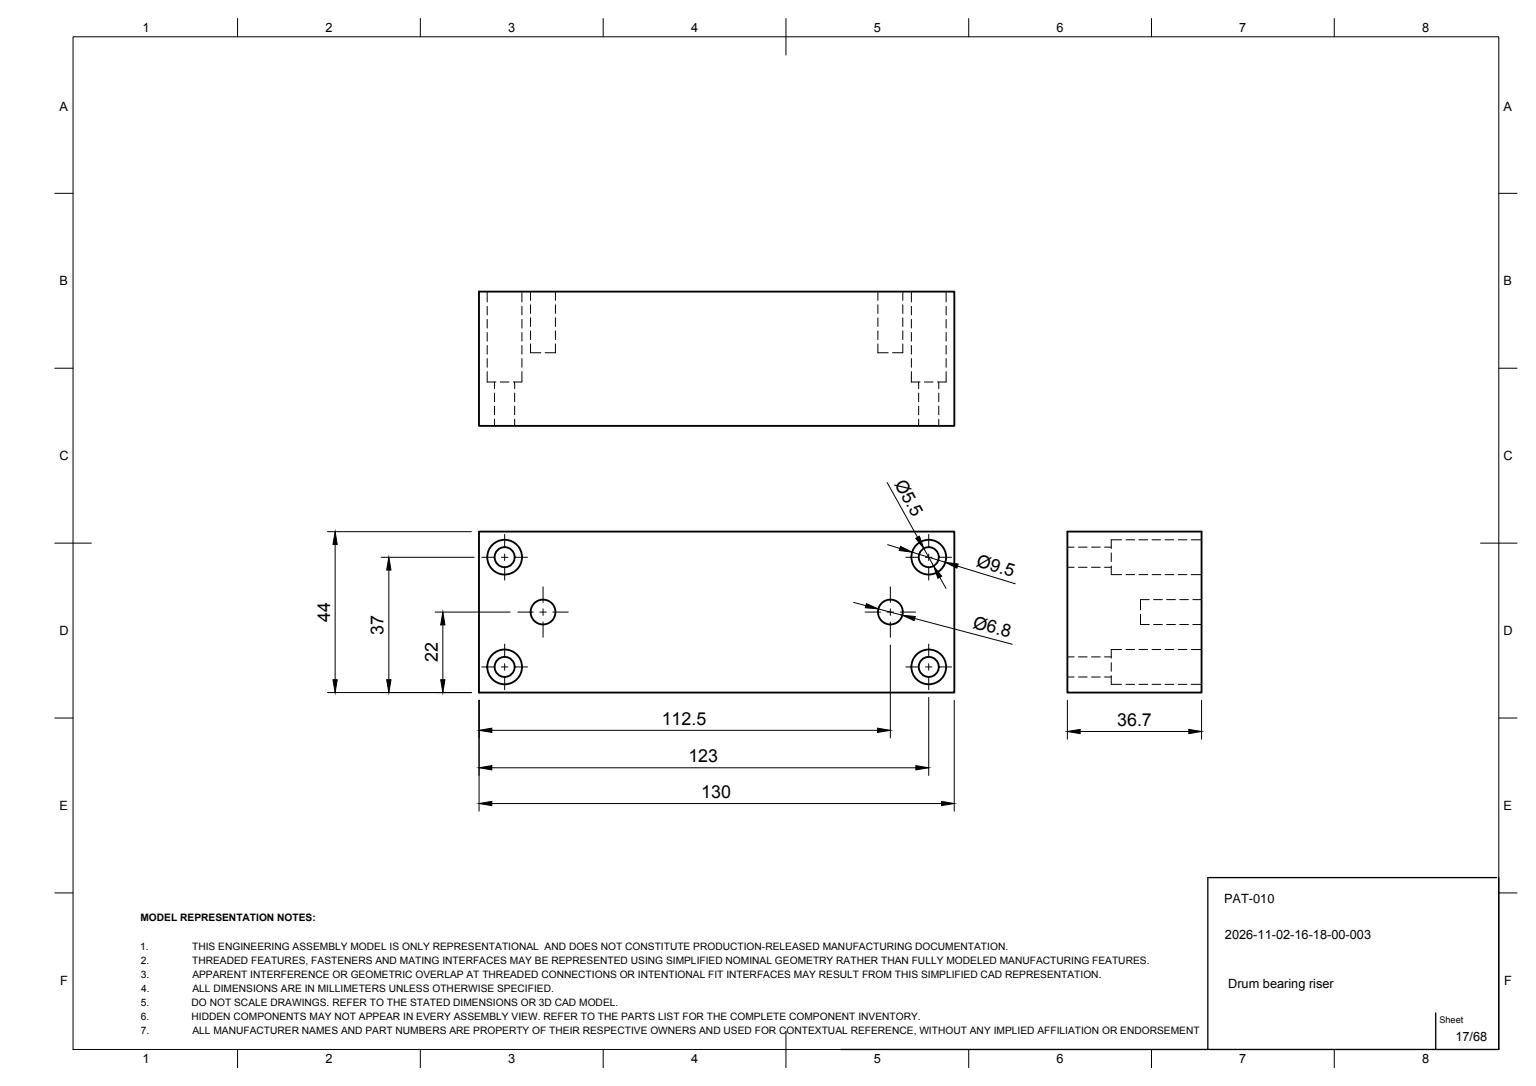
ISO-10303-21;
HEADER;
/* Generated by software containing ST-Developer
 * from STEP Tools, Inc. (www.steptools.com) 
 */

FILE_DESCRIPTION(
/* description */ ('Belt conveyor head drive unit'),
/* implementation_level */ '2;1');

FILE_NAME(
/* name */ 'Drum bearing riser.step',
/* time_stamp */ '2026-10-28T03:26:19-07:00',
/* author */ (''),
/* organization */ (''),
/* preprocessor_version */ 'ST-DEVELOPER v20.2',
/* originating_system */ 'Autodesk Translation Framework v15.17.0.0',
/* authorisation */ '');

FILE_SCHEMA (('AUTOMOTIVE_DESIGN { 1 0 10303 214 3 1 1 }'));
ENDSEC;

DATA;
#10=MECHANICAL_DESIGN_GEOMETRIC_PRESENTATION_REPRESENTATION('',(#863),#27069);
#725=SHAPE_REPRESENTATION_RELATIONSHIP('SRR','None',#27369,#794);
#794=ADVANCED_BREP_SHAPE_REPRESENTATION('',(#948),#27011);
#863=STYLED_ITEM('',(#27797),#948);
#948=MANIFOLD_SOLID_BREP('Body1',#13728);
#1093=FACE_BOUND('',#2714,.T.);
#1094=FACE_BOUND('',#2718,.T.);
#1095=FACE_BOUND('',#2722,.T.);
#1096=FACE_BOUND('',#2726,.T.);
#1097=FACE_BOUND('',#2737,.T.);
#1098=FACE_BOUND('',#2738,.T.);
#1099=FACE_BOUND('',#2739,.T.);
#1100=FACE_BOUND('',#2740,.T.);
#1101=FACE_BOUND('',#2741,.T.);
#1102=FACE_BOUND('',#2742,.T.);
#1103=FACE_BOUND('',#2744,.T.);
#1104=FACE_BOUND('',#2745,.T.);
#1105=FACE_BOUND('',#2746,.T.);
#1106=FACE_BOUND('',#2747,.T.);
#1373=PLANE('',#14998);
#1374=PLANE('',#15005);
#1375=PLANE('',#15012);
#1376=PLANE('',#15019);
#1377=PLANE('',#15026);
#1378=PLANE('',#15030);
#1379=PLANE('',#15031);
#1380=PLANE('',#15032);
#1381=PLANE('',#15033);
#1382=PLANE('',#15034);
#1383=PLANE('',#15035);
#1384=PLANE('',#15036);
#1831=FACE_OUTER_BOUND('',#2712,.T.);
#1832=FACE_OUTER_BOUND('',#2713,.T.);
#1833=FACE_OUTER_BOUND('',#2715,.T.);
#1834=FACE_OUTER_BOUND('',#2716,.T.);
#1835=FACE_OUTER_BOUND('',#2717,.T.);
#1836=FACE_OUTER_BOUND('',#2719,.T.);
#1837=FACE_OUTER_BOUND('',#2720,.T.);
#1838=FACE_OUTER_BOUND('',#2721,.T.);
#1839=FACE_OUTER_BOUND('',#2723,.T.);
#1840=FACE_OUTER_BOUND('',#2724,.T.);
#1841=FACE_OUTER_BOUND('',#2725,.T.);
#1842=FACE_OUTER_BOUND('',#2727,.T.);
#1843=FACE_OUTER_BOUND('',#2728,.T.);
#1844=FACE_OUTER_BOUND('',#2729,.T.);
#1845=FACE_OUTER_BOUND('',#2730,.T.);
#1846=FACE_OUTER_BOUND('',#2731,.T.);
#1847=FACE_OUTER_BOUND('',#2732,.T.);
#1848=FACE_OUTER_BOUND('',#2733,.T.);
#1849=FACE_OUTER_BOUND('',#2734,.T.);
#1850=FACE_OUTER_BOUND('',#2735,.T.);
#1851=FACE_OUTER_BOUND('',#2736,.T.);
#1852=FACE_OUTER_BOUND('',#2743,.T.);
#2712=EDGE_LOOP('',(#9864,#9865,#9866,#9867));
#2713=EDGE_LOOP('',(#9868));
#2714=EDGE_LOOP('',(#9869));
#2715=EDGE_LOOP('',(#9870,#9871,#9872,#9873));
#2716=EDGE_LOOP('',(#9874,#9875,#9876,#9877));
#2717=EDGE_LOOP('',(#9878));
#2718=EDGE_LOOP('',(#9879));
#2719=EDGE_LOOP('',(#9880,#9881,#9882,#9883));
#2720=EDGE_LOOP('',(#9884,#9885,#9886,#9887));
#2721=EDGE_LOOP('',(#9888));
#2722=EDGE_LOOP('',(#9889));
#2723=EDGE_LOOP('',(#9890,#9891,#9892,#9893));
#2724=EDGE_LOOP('',(#9894,#9895,#9896,#9897));
#2725=EDGE_LOOP('',(#9898));
#2726=EDGE_LOOP('',(#9899));
#2727=EDGE_LOOP('',(#9900,#9901,#9902,#9903));
#2728=EDGE_LOOP('',(#9904,#9905,#9906,#9907));
#2729=EDGE_LOOP('',(#9908));
#2730=EDGE_LOOP('',(#9909,#9910,#9911,#9912));
#2731=EDGE_LOOP('',(#9913));
#2732=EDGE_LOOP('',(#9914,#9915,#9916,#9917));
#2733=EDGE_LOOP('',(#9918,#9919,#9920,#9921));
#2734=EDGE_LOOP('',(#9922,#9923,#9924,#9925));
#2735=EDGE_LOOP('',(#9926,#9927,#9928,#9929));
#2736=EDGE_LOOP('',(#9930,#9931,#9932,#9933));
#2737=EDGE_LOOP('',(#9934));
#2738=EDGE_LOOP('',(#9935));
#2739=EDGE_LOOP('',(#9936));
#2740=EDGE_LOOP('',(#9937));
#2741=EDGE_LOOP('',(#9938));
#2742=EDGE_LOOP('',(#9939));
#2743=EDGE_LOOP('',(#9940,#9941,#9942,#9943));
#2744=EDGE_LOOP('',(#9944));
#2745=EDGE_LOOP('',(#9945));
#2746=EDGE_LOOP('',(#9946));
#2747=EDGE_LOOP('',(#9947));
#3735=LINE('',#21946,#4527);
#3736=LINE('',#21954,#4528);
#3737=LINE('',#21959,#4529);
#3738=LINE('',#21967,#4530);
#3739=LINE('',#21972,#4531);
#3740=LINE('',#21980,#4532);
#3741=LINE('',#21985,#4533);
#3742=LINE('',#21993,#4534);
#3743=LINE('',#21998,#4535);
#3744=LINE('',#22005,#4536);
#3745=LINE('',#22011,#4537);
#3746=LINE('',#22013,#4538);
#3747=LINE('',#22015,#4539);
#3748=LINE('',#22016,#4540);
#3749=LINE('',#22019,#4541);
#3750=LINE('',#22021,#4542);
#3751=LINE('',#22022,#4543);
#3752=LINE('',#22025,#4544);
#3753=LINE('',#22027,#4545);
#3754=LINE('',#22028,#4546);
#3755=LINE('',#22030,#4547);
#3756=LINE('',#22031,#4548);
#4527=VECTOR('',#17541,0.475);
#4528=VECTOR('',#17552,0.275);
#4529=VECTOR('',#17557,0.475);
#4530=VECTOR('',#17568,0.275);
#4531=VECTOR('',#17573,0.475);
#4532=VECTOR('',#17584,0.275);
#4533=VECTOR('',#17589,0.475);
#4534=VECTOR('',#17600,0.275);
#4535=VECTOR('',#17605,0.34);
#4536=VECTOR('',#17614,0.34);
#4537=VECTOR('',#17621,1.);
#4538=VECTOR('',#17622,1.);
#4539=VECTOR('',#17623,1.);
#4540=VECTOR('',#17624,1.);
#4541=VECTOR('',#17627,1.);
#4542=VECTOR('',#17628,1.);
#4543=VECTOR('',#17629,1.);
#4544=VECTOR('',#17632,1.);
#4545=VECTOR('',#17633,1.);
#4546=VECTOR('',#17634,1.);
#4547=VECTOR('',#17637,1.);
#4548=VECTOR('',#17638,1.);
#5298=CIRCLE('',#14996,0.475);
#5299=CIRCLE('',#14997,0.475);
#5300=CIRCLE('',#14999,0.275);
#5301=CIRCLE('',#15001,0.275);
#5302=CIRCLE('',#15003,0.475);
#5303=CIRCLE('',#15004,0.475);
#5304=CIRCLE('',#15006,0.275);
#5305=CIRCLE('',#15008,0.275);
#5306=CIRCLE('',#15010,0.475);
#5307=CIRCLE('',#15011,0.475);
#5308=CIRCLE('',#15013,0.275);
#5309=CIRCLE('',#15015,0.275);
#5310=CIRCLE('',#15017,0.475);
#5311=CIRCLE('',#15018,0.475);
#5312=CIRCLE('',#15020,0.275);
#5313=CIRCLE('',#15022,0.275);
#5314=CIRCLE('',#15024,0.34);
#5315=CIRCLE('',#15025,0.34);
#5316=CIRCLE('',#15028,0.34);
#5317=CIRCLE('',#15029,0.34);
#6255=VERTEX_POINT('',#21943);
#6256=VERTEX_POINT('',#21945);
#6257=VERTEX_POINT('',#21949);
#6258=VERTEX_POINT('',#21952);
#6259=VERTEX_POINT('',#21956);
#6260=VERTEX_POINT('',#21958);
#6261=VERTEX_POINT('',#21962);
#6262=VERTEX_POINT('',#21965);
#6263=VERTEX_POINT('',#21969);
#6264=VERTEX_POINT('',#21971);
#6265=VERTEX_POINT('',#21975);
#6266=VERTEX_POINT('',#21978);
#6267=VERTEX_POINT('',#21982);
#6268=VERTEX_POINT('',#21984);
#6269=VERTEX_POINT('',#21988);
#6270=VERTEX_POINT('',#21991);
#6271=VERTEX_POINT('',#21995);
#6272=VERTEX_POINT('',#21997);
#6273=VERTEX_POINT('',#22002);
#6274=VERTEX_POINT('',#22004);
#6275=VERTEX_POINT('',#22009);
#6276=VERTEX_POINT('',#22010);
#6277=VERTEX_POINT('',#22012);
#6278=VERTEX_POINT('',#22014);
#6279=VERTEX_POINT('',#22018);
#6280=VERTEX_POINT('',#22020);
#6281=VERTEX_POINT('',#22024);
#6282=VERTEX_POINT('',#22026);
#7624=EDGE_CURVE('',#6255,#6255,#5298,.T.);
#7625=EDGE_CURVE('',#6255,#6256,#3735,.T.);
#7626=EDGE_CURVE('',#6256,#6256,#5299,.T.);
#7627=EDGE_CURVE('',#6257,#6257,#5300,.T.);
#7628=EDGE_CURVE('',#6258,#6258,#5301,.T.);
#7629=EDGE_CURVE('',#6258,#6257,#3736,.T.);
#7630=EDGE_CURVE('',#6259,#6259,#5302,.T.);
#7631=EDGE_CURVE('',#6259,#6260,#3737,.T.);
#7632=EDGE_CURVE('',#6260,#6260,#5303,.T.);
#7633=EDGE_CURVE('',#6261,#6261,#5304,.T.);
#7634=EDGE_CURVE('',#6262,#6262,#5305,.T.);
#7635=EDGE_CURVE('',#6262,#6261,#3738,.T.);
#7636=EDGE_CURVE('',#6263,#6263,#5306,.T.);
#7637=EDGE_CURVE('',#6263,#6264,#3739,.T.);
#7638=EDGE_CURVE('',#6264,#6264,#5307,.T.);
#7639=EDGE_CURVE('',#6265,#6265,#5308,.T.);
#7640=EDGE_CURVE('',#6266,#6266,#5309,.T.);
#7641=EDGE_CURVE('',#6266,#6265,#3740,.T.);
#7642=EDGE_CURVE('',#6267,#6267,#5310,.T.);
#7643=EDGE_CURVE('',#6267,#6268,#3741,.T.);
#7644=EDGE_CURVE('',#6268,#6268,#5311,.T.);
#7645=EDGE_CURVE('',#6269,#6269,#5312,.T.);
#7646=EDGE_CURVE('',#6270,#6270,#5313,.T.);
#7647=EDGE_CURVE('',#6270,#6269,#3742,.T.);
#7648=EDGE_CURVE('',#6271,#6271,#5314,.T.);
#7649=EDGE_CURVE('',#6271,#6272,#3743,.T.);
#7650=EDGE_CURVE('',#6272,#6272,#5315,.T.);
#7651=EDGE_CURVE('',#6273,#6273,#5316,.T.);
#7652=EDGE_CURVE('',#6273,#6274,#3744,.T.);
#7653=EDGE_CURVE('',#6274,#6274,#5317,.T.);
#7654=EDGE_CURVE('',#6275,#6276,#3745,.T.);
#7655=EDGE_CURVE('',#6276,#6277,#3746,.T.);
#7656=EDGE_CURVE('',#6278,#6277,#3747,.T.);
#7657=EDGE_CURVE('',#6275,#6278,#3748,.T.);
#7658=EDGE_CURVE('',#6279,#6275,#3749,.T.);
#7659=EDGE_CURVE('',#6280,#6278,#3750,.T.);
#7660=EDGE_CURVE('',#6279,#6280,#3751,.T.);
#7661=EDGE_CURVE('',#6281,#6279,#3752,.T.);
#7662=EDGE_CURVE('',#6282,#6280,#3753,.T.);
#7663=EDGE_CURVE('',#6281,#6282,#3754,.T.);
#7664=EDGE_CURVE('',#6276,#6281,#3755,.T.);
#7665=EDGE_CURVE('',#6277,#6282,#3756,.T.);
#9864=ORIENTED_EDGE('',*,*,#7624,.F.);
#9865=ORIENTED_EDGE('',*,*,#7625,.T.);
#9866=ORIENTED_EDGE('',*,*,#7626,.F.);
#9867=ORIENTED_EDGE('',*,*,#7625,.F.);
#9868=ORIENTED_EDGE('',*,*,#7624,.T.);
#9869=ORIENTED_EDGE('',*,*,#7627,.F.);
#9870=ORIENTED_EDGE('',*,*,#7628,.F.);
#9871=ORIENTED_EDGE('',*,*,#7629,.T.);
#9872=ORIENTED_EDGE('',*,*,#7627,.T.);
#9873=ORIENTED_EDGE('',*,*,#7629,.F.);
#9874=ORIENTED_EDGE('',*,*,#7630,.F.);
#9875=ORIENTED_EDGE('',*,*,#7631,.T.);
#9876=ORIENTED_EDGE('',*,*,#7632,.F.);
#9877=ORIENTED_EDGE('',*,*,#7631,.F.);
#9878=ORIENTED_EDGE('',*,*,#7630,.T.);
#9879=ORIENTED_EDGE('',*,*,#7633,.F.);
#9880=ORIENTED_EDGE('',*,*,#7634,.F.);
#9881=ORIENTED_EDGE('',*,*,#7635,.T.);
#9882=ORIENTED_EDGE('',*,*,#7633,.T.);
#9883=ORIENTED_EDGE('',*,*,#7635,.F.);
#9884=ORIENTED_EDGE('',*,*,#7636,.F.);
#9885=ORIENTED_EDGE('',*,*,#7637,.T.);
#9886=ORIENTED_EDGE('',*,*,#7638,.F.);
#9887=ORIENTED_EDGE('',*,*,#7637,.F.);
#9888=ORIENTED_EDGE('',*,*,#7636,.T.);
#9889=ORIENTED_EDGE('',*,*,#7639,.F.);
#9890=ORIENTED_EDGE('',*,*,#7640,.F.);
#9891=ORIENTED_EDGE('',*,*,#7641,.T.);
#9892=ORIENTED_EDGE('',*,*,#7639,.T.);
#9893=ORIENTED_EDGE('',*,*,#7641,.F.);
#9894=ORIENTED_EDGE('',*,*,#7642,.F.);
#9895=ORIENTED_EDGE('',*,*,#7643,.T.);
#9896=ORIENTED_EDGE('',*,*,#7644,.F.);
#9897=ORIENTED_EDGE('',*,*,#7643,.F.);
#9898=ORIENTED_EDGE('',*,*,#7642,.T.);
#9899=ORIENTED_EDGE('',*,*,#7645,.F.);
#9900=ORIENTED_EDGE('',*,*,#7646,.F.);
#9901=ORIENTED_EDGE('',*,*,#7647,.T.);
#9902=ORIENTED_EDGE('',*,*,#7645,.T.);
#9903=ORIENTED_EDGE('',*,*,#7647,.F.);
#9904=ORIENTED_EDGE('',*,*,#7648,.F.);
#9905=ORIENTED_EDGE('',*,*,#7649,.T.);
#9906=ORIENTED_EDGE('',*,*,#7650,.F.);
#9907=ORIENTED_EDGE('',*,*,#7649,.F.);
#9908=ORIENTED_EDGE('',*,*,#7648,.T.);
#9909=ORIENTED_EDGE('',*,*,#7651,.F.);
#9910=ORIENTED_EDGE('',*,*,#7652,.T.);
#9911=ORIENTED_EDGE('',*,*,#7653,.F.);
#9912=ORIENTED_EDGE('',*,*,#7652,.F.);
#9913=ORIENTED_EDGE('',*,*,#7651,.T.);
#9914=ORIENTED_EDGE('',*,*,#7654,.T.);
#9915=ORIENTED_EDGE('',*,*,#7655,.T.);
#9916=ORIENTED_EDGE('',*,*,#7656,.F.);
#9917=ORIENTED_EDGE('',*,*,#7657,.F.);
#9918=ORIENTED_EDGE('',*,*,#7658,.T.);
#9919=ORIENTED_EDGE('',*,*,#7657,.T.);
#9920=ORIENTED_EDGE('',*,*,#7659,.F.);
#9921=ORIENTED_EDGE('',*,*,#7660,.F.);
#9922=ORIENTED_EDGE('',*,*,#7661,.T.);
#9923=ORIENTED_EDGE('',*,*,#7660,.T.);
#9924=ORIENTED_EDGE('',*,*,#7662,.F.);
#9925=ORIENTED_EDGE('',*,*,#7663,.F.);
#9926=ORIENTED_EDGE('',*,*,#7664,.T.);
#9927=ORIENTED_EDGE('',*,*,#7663,.T.);
#9928=ORIENTED_EDGE('',*,*,#7665,.F.);
#9929=ORIENTED_EDGE('',*,*,#7655,.F.);
#9930=ORIENTED_EDGE('',*,*,#7665,.T.);
#9931=ORIENTED_EDGE('',*,*,#7662,.T.);
#9932=ORIENTED_EDGE('',*,*,#7659,.T.);
#9933=ORIENTED_EDGE('',*,*,#7656,.T.);
#9934=ORIENTED_EDGE('',*,*,#7626,.T.);
#9935=ORIENTED_EDGE('',*,*,#7632,.T.);
#9936=ORIENTED_EDGE('',*,*,#7638,.T.);
#9937=ORIENTED_EDGE('',*,*,#7644,.T.);
#9938=ORIENTED_EDGE('',*,*,#7650,.T.);
#9939=ORIENTED_EDGE('',*,*,#7653,.T.);
#9940=ORIENTED_EDGE('',*,*,#7664,.F.);
#9941=ORIENTED_EDGE('',*,*,#7654,.F.);
#9942=ORIENTED_EDGE('',*,*,#7658,.F.);
#9943=ORIENTED_EDGE('',*,*,#7661,.F.);
#9944=ORIENTED_EDGE('',*,*,#7628,.T.);
#9945=ORIENTED_EDGE('',*,*,#7634,.T.);
#9946=ORIENTED_EDGE('',*,*,#7640,.T.);
#9947=ORIENTED_EDGE('',*,*,#7646,.T.);
#12634=CYLINDRICAL_SURFACE('',#14995,0.475);
#12635=CYLINDRICAL_SURFACE('',#15000,0.275);
#12636=CYLINDRICAL_SURFACE('',#15002,0.475);
#12637=CYLINDRICAL_SURFACE('',#15007,0.275);
#12638=CYLINDRICAL_SURFACE('',#15009,0.475);
#12639=CYLINDRICAL_SURFACE('',#15014,0.275);
#12640=CYLINDRICAL_SURFACE('',#15016,0.475);
#12641=CYLINDRICAL_SURFACE('',#15021,0.275);
#12642=CYLINDRICAL_SURFACE('',#15023,0.34);
#12643=CYLINDRICAL_SURFACE('',#15027,0.34);
#13110=ADVANCED_FACE('',(#1831),#12634,.F.);
#13111=ADVANCED_FACE('',(#1832,#1093),#1373,.T.);
#13112=ADVANCED_FACE('',(#1833),#12635,.F.);
#13113=ADVANCED_FACE('',(#1834),#12636,.F.);
#13114=ADVANCED_FACE('',(#1835,#1094),#1374,.T.);
#13115=ADVANCED_FACE('',(#1836),#12637,.F.);
#13116=ADVANCED_FACE('',(#1837),#12638,.F.);
#13117=ADVANCED_FACE('',(#1838,#1095),#1375,.T.);
#13118=ADVANCED_FACE('',(#1839),#12639,.F.);
#13119=ADVANCED_FACE('',(#1840),#12640,.F.);
#13120=ADVANCED_FACE('',(#1841,#1096),#1376,.T.);
#13121=ADVANCED_FACE('',(#1842),#12641,.F.);
#13122=ADVANCED_FACE('',(#1843),#12642,.F.);
#13123=ADVANCED_FACE('',(#1844),#1377,.T.);
#13124=ADVANCED_FACE('',(#1845),#12643,.F.);
#13125=ADVANCED_FACE('',(#1846),#1378,.T.);
#13126=ADVANCED_FACE('',(#1847),#1379,.T.);
#13127=ADVANCED_FACE('',(#1848),#1380,.T.);
#13128=ADVANCED_FACE('',(#1849),#1381,.T.);
#13129=ADVANCED_FACE('',(#1850),#1382,.T.);
#13130=ADVANCED_FACE('',(#1851,#1097,#1098,#1099,#1100,#1101,#1102),#1383,
 .T.);
#13131=ADVANCED_FACE('',(#1852,#1103,#1104,#1105,#1106),#1384,.F.);
#13728=CLOSED_SHELL('',(#13110,#13111,#13112,#13113,#13114,#13115,#13116,
#13117,#13118,#13119,#13120,#13121,#13122,#13123,#13124,#13125,#13126,#13127,
#13128,#13129,#13130,#13131));
#14994=AXIS2_PLACEMENT_3D('',#21941,#17535,#17536);
#14995=AXIS2_PLACEMENT_3D('',#21942,#17537,#17538);
#14996=AXIS2_PLACEMENT_3D('',#21944,#17539,#17540);
#14997=AXIS2_PLACEMENT_3D('',#21947,#17542,#17543);
#14998=AXIS2_PLACEMENT_3D('',#21948,#17544,#17545);
#14999=AXIS2_PLACEMENT_3D('',#21950,#17546,#17547);
#15000=AXIS2_PLACEMENT_3D('',#21951,#17548,#17549);
#15001=AXIS2_PLACEMENT_3D('',#21953,#17550,#17551);
#15002=AXIS2_PLACEMENT_3D('',#21955,#17553,#17554);
#15003=AXIS2_PLACEMENT_3D('',#21957,#17555,#17556);
#15004=AXIS2_PLACEMENT_3D('',#21960,#17558,#17559);
#15005=AXIS2_PLACEMENT_3D('',#21961,#17560,#17561);
#15006=AXIS2_PLACEMENT_3D('',#21963,#17562,#17563);
#15007=AXIS2_PLACEMENT_3D('',#21964,#17564,#17565);
#15008=AXIS2_PLACEMENT_3D('',#21966,#17566,#17567);
#15009=AXIS2_PLACEMENT_3D('',#21968,#17569,#17570);
#15010=AXIS2_PLACEMENT_3D('',#21970,#17571,#17572);
#15011=AXIS2_PLACEMENT_3D('',#21973,#17574,#17575);
#15012=AXIS2_PLACEMENT_3D('',#21974,#17576,#17577);
#15013=AXIS2_PLACEMENT_3D('',#21976,#17578,#17579);
#15014=AXIS2_PLACEMENT_3D('',#21977,#17580,#17581);
#15015=AXIS2_PLACEMENT_3D('',#21979,#17582,#17583);
#15016=AXIS2_PLACEMENT_3D('',#21981,#17585,#17586);
#15017=AXIS2_PLACEMENT_3D('',#21983,#17587,#17588);
#15018=AXIS2_PLACEMENT_3D('',#21986,#17590,#17591);
#15019=AXIS2_PLACEMENT_3D('',#21987,#17592,#17593);
#15020=AXIS2_PLACEMENT_3D('',#21989,#17594,#17595);
#15021=AXIS2_PLACEMENT_3D('',#21990,#17596,#17597);
#15022=AXIS2_PLACEMENT_3D('',#21992,#17598,#17599);
#15023=AXIS2_PLACEMENT_3D('',#21994,#17601,#17602);
#15024=AXIS2_PLACEMENT_3D('',#21996,#17603,#17604);
#15025=AXIS2_PLACEMENT_3D('',#21999,#17606,#17607);
#15026=AXIS2_PLACEMENT_3D('',#22000,#17608,#17609);
#15027=AXIS2_PLACEMENT_3D('',#22001,#17610,#17611);
#15028=AXIS2_PLACEMENT_3D('',#22003,#17612,#17613);
#15029=AXIS2_PLACEMENT_3D('',#22006,#17615,#17616);
#15030=AXIS2_PLACEMENT_3D('',#22007,#17617,#17618);
#15031=AXIS2_PLACEMENT_3D('',#22008,#17619,#17620);
#15032=AXIS2_PLACEMENT_3D('',#22017,#17625,#17626);
#15033=AXIS2_PLACEMENT_3D('',#22023,#17630,#17631);
#15034=AXIS2_PLACEMENT_3D('',#22029,#17635,#17636);
#15035=AXIS2_PLACEMENT_3D('',#22032,#17639,#17640);
#15036=AXIS2_PLACEMENT_3D('',#22033,#17641,#17642);
#17535=DIRECTION('axis',(0.,0.,1.));
#17536=DIRECTION('refdir',(1.,0.,0.));
#17537=DIRECTION('center_axis',(0.,0.,1.));
#17538=DIRECTION('ref_axis',(1.,0.,0.));
#17539=DIRECTION('center_axis',(0.,0.,1.));
#17540=DIRECTION('ref_axis',(1.,0.,0.));
#17541=DIRECTION('',(0.,0.,1.));
#17542=DIRECTION('center_axis',(0.,0.,-1.));
#17543=DIRECTION('ref_axis',(1.,0.,0.));
#17544=DIRECTION('center_axis',(0.,0.,1.));
#17545=DIRECTION('ref_axis',(1.,0.,0.));
#17546=DIRECTION('center_axis',(0.,0.,1.));
#17547=DIRECTION('ref_axis',(1.,0.,0.));
#17548=DIRECTION('center_axis',(0.,0.,1.));
#17549=DIRECTION('ref_axis',(1.,0.,0.));
#17550=DIRECTION('center_axis',(0.,0.,1.));
#17551=DIRECTION('ref_axis',(1.,0.,0.));
#17552=DIRECTION('',(0.,0.,1.));
#17553=DIRECTION('center_axis',(0.,0.,1.));
#17554=DIRECTION('ref_axis',(1.,0.,0.));
#17555=DIRECTION('center_axis',(0.,0.,1.));
#17556=DIRECTION('ref_axis',(1.,0.,0.));
#17557=DIRECTION('',(0.,0.,1.));
#17558=DIRECTION('center_axis',(0.,0.,-1.));
#17559=DIRECTION('ref_axis',(1.,0.,0.));
#17560=DIRECTION('center_axis',(0.,0.,1.));
#17561=DIRECTION('ref_axis',(1.,0.,0.));
#17562=DIRECTION('center_axis',(0.,0.,1.));
#17563=DIRECTION('ref_axis',(1.,0.,0.));
#17564=DIRECTION('center_axis',(0.,0.,1.));
#17565=DIRECTION('ref_axis',(1.,0.,0.));
#17566=DIRECTION('center_axis',(0.,0.,1.));
#17567=DIRECTION('ref_axis',(1.,0.,0.));
#17568=DIRECTION('',(0.,0.,1.));
#17569=DIRECTION('center_axis',(0.,0.,1.));
#17570=DIRECTION('ref_axis',(1.,0.,0.));
#17571=DIRECTION('center_axis',(0.,0.,1.));
#17572=DIRECTION('ref_axis',(1.,0.,0.));
#17573=DIRECTION('',(0.,0.,1.));
#17574=DIRECTION('center_axis',(0.,0.,-1.));
#17575=DIRECTION('ref_axis',(1.,0.,0.));
#17576=DIRECTION('center_axis',(0.,0.,1.));
#17577=DIRECTION('ref_axis',(1.,0.,0.));
#17578=DIRECTION('center_axis',(0.,0.,1.));
#17579=DIRECTION('ref_axis',(1.,0.,0.));
#17580=DIRECTION('center_axis',(0.,0.,1.));
#17581=DIRECTION('ref_axis',(1.,0.,0.));
#17582=DIRECTION('center_axis',(0.,0.,1.));
#17583=DIRECTION('ref_axis',(1.,0.,0.));
#17584=DIRECTION('',(0.,0.,1.));
#17585=DIRECTION('center_axis',(0.,0.,1.));
#17586=DIRECTION('ref_axis',(1.,0.,0.));
#17587=DIRECTION('center_axis',(0.,0.,1.));
#17588=DIRECTION('ref_axis',(1.,0.,0.));
#17589=DIRECTION('',(0.,0.,1.));
#17590=DIRECTION('center_axis',(0.,0.,-1.));
#17591=DIRECTION('ref_axis',(1.,0.,0.));
#17592=DIRECTION('center_axis',(0.,0.,1.));
#17593=DIRECTION('ref_axis',(1.,0.,0.));
#17594=DIRECTION('center_axis',(0.,0.,1.));
#17595=DIRECTION('ref_axis',(1.,0.,0.));
#17596=DIRECTION('center_axis',(0.,0.,1.));
#17597=DIRECTION('ref_axis',(1.,0.,0.));
#17598=DIRECTION('center_axis',(0.,0.,1.));
#17599=DIRECTION('ref_axis',(1.,0.,0.));
#17600=DIRECTION('',(0.,0.,1.));
#17601=DIRECTION('center_axis',(0.,0.,1.));
#17602=DIRECTION('ref_axis',(1.,0.,0.));
#17603=DIRECTION('center_axis',(0.,0.,1.));
#17604=DIRECTION('ref_axis',(1.,0.,0.));
#17605=DIRECTION('',(0.,0.,1.));
#17606=DIRECTION('center_axis',(0.,0.,-1.));
#17607=DIRECTION('ref_axis',(1.,0.,0.));
#17608=DIRECTION('center_axis',(0.,0.,1.));
#17609=DIRECTION('ref_axis',(1.,0.,0.));
#17610=DIRECTION('center_axis',(0.,0.,1.));
#17611=DIRECTION('ref_axis',(1.,0.,0.));
#17612=DIRECTION('center_axis',(0.,0.,1.));
#17613=DIRECTION('ref_axis',(1.,0.,0.));
#17614=DIRECTION('',(0.,0.,1.));
#17615=DIRECTION('center_axis',(0.,0.,-1.));
#17616=DIRECTION('ref_axis',(1.,0.,0.));
#17617=DIRECTION('center_axis',(0.,0.,1.));
#17618=DIRECTION('ref_axis',(1.,0.,0.));
#17619=DIRECTION('center_axis',(0.,1.,0.));
#17620=DIRECTION('ref_axis',(-1.,0.,0.));
#17621=DIRECTION('',(-1.,0.,0.));
#17622=DIRECTION('',(0.,0.,1.));
#17623=DIRECTION('',(-1.,0.,0.));
#17624=DIRECTION('',(0.,0.,1.));
#17625=DIRECTION('center_axis',(1.,0.,0.));
#17626=DIRECTION('ref_axis',(0.,1.,0.));
#17627=DIRECTION('',(0.,1.,0.));
#17628=DIRECTION('',(0.,1.,0.));
#17629=DIRECTION('',(0.,0.,1.));
#17630=DIRECTION('center_axis',(0.,-1.,0.));
#17631=DIRECTION('ref_axis',(1.,0.,0.));
#17632=DIRECTION('',(1.,0.,0.));
#17633=DIRECTION('',(1.,0.,0.));
#17634=DIRECTION('',(0.,0.,1.));
#17635=DIRECTION('center_axis',(-1.,0.,0.));
#17636=DIRECTION('ref_axis',(0.,-1.,0.));
#17637=DIRECTION('',(0.,-1.,0.));
#17638=DIRECTION('',(0.,-1.,0.));
#17639=DIRECTION('center_axis',(0.,0.,1.));
#17640=DIRECTION('ref_axis',(1.,0.,0.));
#17641=DIRECTION('center_axis',(0.,0.,1.));
#17642=DIRECTION('ref_axis',(1.,0.,0.));
#21941=CARTESIAN_POINT('',(0.,0.,0.));
#21942=CARTESIAN_POINT('Origin',(12.7709100301812,5.5,1.2));
#21943=CARTESIAN_POINT('',(12.2959100301812,5.5,1.2));
#21944=CARTESIAN_POINT('Origin',(12.7709100301812,5.5,1.2));
#21945=CARTESIAN_POINT('',(12.2959100301812,5.5,3.67));
#21946=CARTESIAN_POINT('',(12.2959100301812,5.5,1.2));
#21947=CARTESIAN_POINT('Origin',(12.7709100301812,5.5,3.67));
#21948=CARTESIAN_POINT('Origin',(12.7709100301812,5.5,1.2));
#21949=CARTESIAN_POINT('',(12.4959100301812,5.5,1.2));
#21950=CARTESIAN_POINT('Origin',(12.7709100301812,5.5,1.2));
#21951=CARTESIAN_POINT('Origin',(12.7709100301812,5.5,-0.1));
#21952=CARTESIAN_POINT('',(12.4959100301812,5.5,0.));
#21953=CARTESIAN_POINT('Origin',(12.7709100301812,5.5,0.));
#21954=CARTESIAN_POINT('',(12.4959100301812,5.5,-0.1));
#21955=CARTESIAN_POINT('Origin',(12.7709100301812,2.5,1.2));
#21956=CARTESIAN_POINT('',(12.2959100301812,2.5,1.2));
#21957=CARTESIAN_POINT('Origin',(12.7709100301812,2.5,1.2));
#21958=CARTESIAN_POINT('',(12.2959100301812,2.5,3.67));
#21959=CARTESIAN_POINT('',(12.2959100301812,2.5,1.2));
#21960=CARTESIAN_POINT('Origin',(12.7709100301812,2.5,3.67));
#21961=CARTESIAN_POINT('Origin',(12.7709100301812,2.5,1.2));
#21962=CARTESIAN_POINT('',(12.4959100301812,2.5,1.2));
#21963=CARTESIAN_POINT('Origin',(12.7709100301812,2.5,1.2));
#21964=CARTESIAN_POINT('Origin',(12.7709100301812,2.5,-0.1));
#21965=CARTESIAN_POINT('',(12.4959100301812,2.5,0.));
#21966=CARTESIAN_POINT('Origin',(12.7709100301812,2.5,0.));
#21967=CARTESIAN_POINT('',(12.4959100301812,2.5,-0.1));
#21968=CARTESIAN_POINT('Origin',(1.17091003018116,5.5,1.2));
#21969=CARTESIAN_POINT('',(0.695910030181156,5.5,1.2));
#21970=CARTESIAN_POINT('Origin',(1.17091003018116,5.5,1.2));
#21971=CARTESIAN_POINT('',(0.695910030181156,5.5,3.67));
#21972=CARTESIAN_POINT('',(0.695910030181156,5.5,1.2));
#21973=CARTESIAN_POINT('Origin',(1.17091003018116,5.5,3.67));
#21974=CARTESIAN_POINT('Origin',(1.17091003018116,5.5,1.2));
#21975=CARTESIAN_POINT('',(0.895910030181156,5.5,1.2));
#21976=CARTESIAN_POINT('Origin',(1.17091003018116,5.5,1.2));
#21977=CARTESIAN_POINT('Origin',(1.17091003018116,5.5,-0.1));
#21978=CARTESIAN_POINT('',(0.895910030181156,5.5,0.));
#21979=CARTESIAN_POINT('Origin',(1.17091003018116,5.5,0.));
#21980=CARTESIAN_POINT('',(0.895910030181156,5.5,-0.1));
#21981=CARTESIAN_POINT('Origin',(1.17091003018116,2.5,1.2));
#21982=CARTESIAN_POINT('',(0.695910030181156,2.5,1.2));
#21983=CARTESIAN_POINT('Origin',(1.17091003018116,2.5,1.2));
#21984=CARTESIAN_POINT('',(0.695910030181156,2.5,3.67));
#21985=CARTESIAN_POINT('',(0.695910030181156,2.5,1.2));
#21986=CARTESIAN_POINT('Origin',(1.17091003018116,2.5,3.67));
#21987=CARTESIAN_POINT('Origin',(1.17091003018116,2.5,1.2));
#21988=CARTESIAN_POINT('',(0.895910030181156,2.5,1.2));
#21989=CARTESIAN_POINT('Origin',(1.17091003018116,2.5,1.2));
#21990=CARTESIAN_POINT('Origin',(1.17091003018116,2.5,-0.1));
#21991=CARTESIAN_POINT('',(0.895910030181156,2.5,0.));
#21992=CARTESIAN_POINT('Origin',(1.17091003018116,2.5,0.));
#21993=CARTESIAN_POINT('',(0.895910030181156,2.5,-0.1));
#21994=CARTESIAN_POINT('Origin',(2.22091003018116,4.,2.));
#21995=CARTESIAN_POINT('',(1.88091003018116,4.,2.));
#21996=CARTESIAN_POINT('Origin',(2.22091003018116,4.,2.));
#21997=CARTESIAN_POINT('',(1.88091003018116,4.,3.67));
#21998=CARTESIAN_POINT('',(1.88091003018116,4.,2.));
#21999=CARTESIAN_POINT('Origin',(2.22091003018116,4.,3.67));
#22000=CARTESIAN_POINT('Origin',(2.22091003018116,4.,2.));
#22001=CARTESIAN_POINT('Origin',(11.7209100301812,4.,2.));
#22002=CARTESIAN_POINT('',(11.3809100301812,4.,2.));
#22003=CARTESIAN_POINT('Origin',(11.7209100301812,4.,2.));
#22004=CARTESIAN_POINT('',(11.3809100301812,4.,3.67));
#22005=CARTESIAN_POINT('',(11.3809100301812,4.,2.));
#22006=CARTESIAN_POINT('Origin',(11.7209100301812,4.,3.67));
#22007=CARTESIAN_POINT('Origin',(11.7209100301812,4.,2.));
#22008=CARTESIAN_POINT('Origin',(13.4709100301812,6.2,0.));
#22009=CARTESIAN_POINT('',(13.4709100301812,6.2,0.));
#22010=CARTESIAN_POINT('',(0.470910030181156,6.2,0.));
#22011=CARTESIAN_POINT('',(13.4709100301812,6.2,0.));
#22012=CARTESIAN_POINT('',(0.470910030181156,6.2,3.67));
#22013=CARTESIAN_POINT('',(0.470910030181156,6.2,0.));
#22014=CARTESIAN_POINT('',(13.4709100301812,6.2,3.67));
#22015=CARTESIAN_POINT('',(13.4709100301812,6.2,3.67));
#22016=CARTESIAN_POINT('',(13.4709100301812,6.2,0.));
#22017=CARTESIAN_POINT('Origin',(13.4709100301812,1.8,0.));
#22018=CARTESIAN_POINT('',(13.4709100301812,1.8,0.));
#22019=CARTESIAN_POINT('',(13.4709100301812,1.8,0.));
#22020=CARTESIAN_POINT('',(13.4709100301812,1.8,3.67));
#22021=CARTESIAN_POINT('',(13.4709100301812,1.8,3.67));
#22022=CARTESIAN_POINT('',(13.4709100301812,1.8,0.));
#22023=CARTESIAN_POINT('Origin',(0.470910030181156,1.8,0.));
#22024=CARTESIAN_POINT('',(0.470910030181156,1.8,0.));
#22025=CARTESIAN_POINT('',(0.470910030181156,1.8,0.));
#22026=CARTESIAN_POINT('',(0.470910030181156,1.8,3.67));
#22027=CARTESIAN_POINT('',(0.470910030181156,1.8,3.67));
#22028=CARTESIAN_POINT('',(0.470910030181156,1.8,0.));
#22029=CARTESIAN_POINT('Origin',(0.470910030181156,6.2,0.));
#22030=CARTESIAN_POINT('',(0.470910030181156,6.2,0.));
#22031=CARTESIAN_POINT('',(0.470910030181156,6.2,3.67));
#22032=CARTESIAN_POINT('Origin',(6.97091003018116,4.,3.67));
#22033=CARTESIAN_POINT('Origin',(6.97091003018116,4.,0.));
#26934=UNCERTAINTY_MEASURE_WITH_UNIT(LENGTH_MEASURE(0.001),#27070,
'DISTANCE_ACCURACY_VALUE',
'Maximum model space distance between geometric entities at asserted c
onnectivities');
#26992=UNCERTAINTY_MEASURE_WITH_UNIT(LENGTH_MEASURE(0.001),#27070,
'DISTANCE_ACCURACY_VALUE',
'Maximum model space distance between geometric entities at asserted c
onnectivities');
#27011=(
GEOMETRIC_REPRESENTATION_CONTEXT(3)
GLOBAL_UNCERTAINTY_ASSIGNED_CONTEXT((#26934))
GLOBAL_UNIT_ASSIGNED_CONTEXT((#27070,#27072,#27073))
REPRESENTATION_CONTEXT('','3D')
);
#27069=(
GEOMETRIC_REPRESENTATION_CONTEXT(3)
GLOBAL_UNCERTAINTY_ASSIGNED_CONTEXT((#26992))
GLOBAL_UNIT_ASSIGNED_CONTEXT((#27070,#27072,#27073))
REPRESENTATION_CONTEXT('','3D')
);
#27070=(
LENGTH_UNIT()
NAMED_UNIT(*)
SI_UNIT(.CENTI.,.METRE.)
);
#27072=(
NAMED_UNIT(*)
PLANE_ANGLE_UNIT()
SI_UNIT($,.RADIAN.)
);
#27073=(
NAMED_UNIT(*)
SI_UNIT($,.STERADIAN.)
SOLID_ANGLE_UNIT()
);
#27092=SHAPE_DEFINITION_REPRESENTATION(#27168,#27369);
#27168=PRODUCT_DEFINITION_SHAPE('',$,#27446);
#27369=SHAPE_REPRESENTATION('',(#14994),#27011);
#27427=PRODUCT_DEFINITION_CONTEXT('part definition',#27657,'design');
#27446=PRODUCT_DEFINITION('Drum bearing riser','Drum bearing riser',#27522,
#27427);
#27522=PRODUCT_DEFINITION_FORMATION('',$,#27677);
#27657=APPLICATION_CONTEXT(
'Core Data for Automotive Mechanical Design Process');
#27658=PRODUCT_CONTEXT('part definition',#27657,'mechanical');
#27677=PRODUCT('Drum bearing riser','Drum bearing riser',
'Drum bearing riser',(#27658));
#27791=COLOUR_RGB('Grey',0.48,0.52,0.57);
#27792=FILL_AREA_STYLE_COLOUR('',#27791);
#27793=FILL_AREA_STYLE('',(#27792));
#27794=SURFACE_STYLE_FILL_AREA(#27793);
#27795=SURFACE_SIDE_STYLE('',(#27794));
#27796=SURFACE_STYLE_USAGE(.BOTH.,#27795);
#27797=PRESENTATION_STYLE_ASSIGNMENT((#27796));
ENDSEC;
END-ISO-10303-21;
